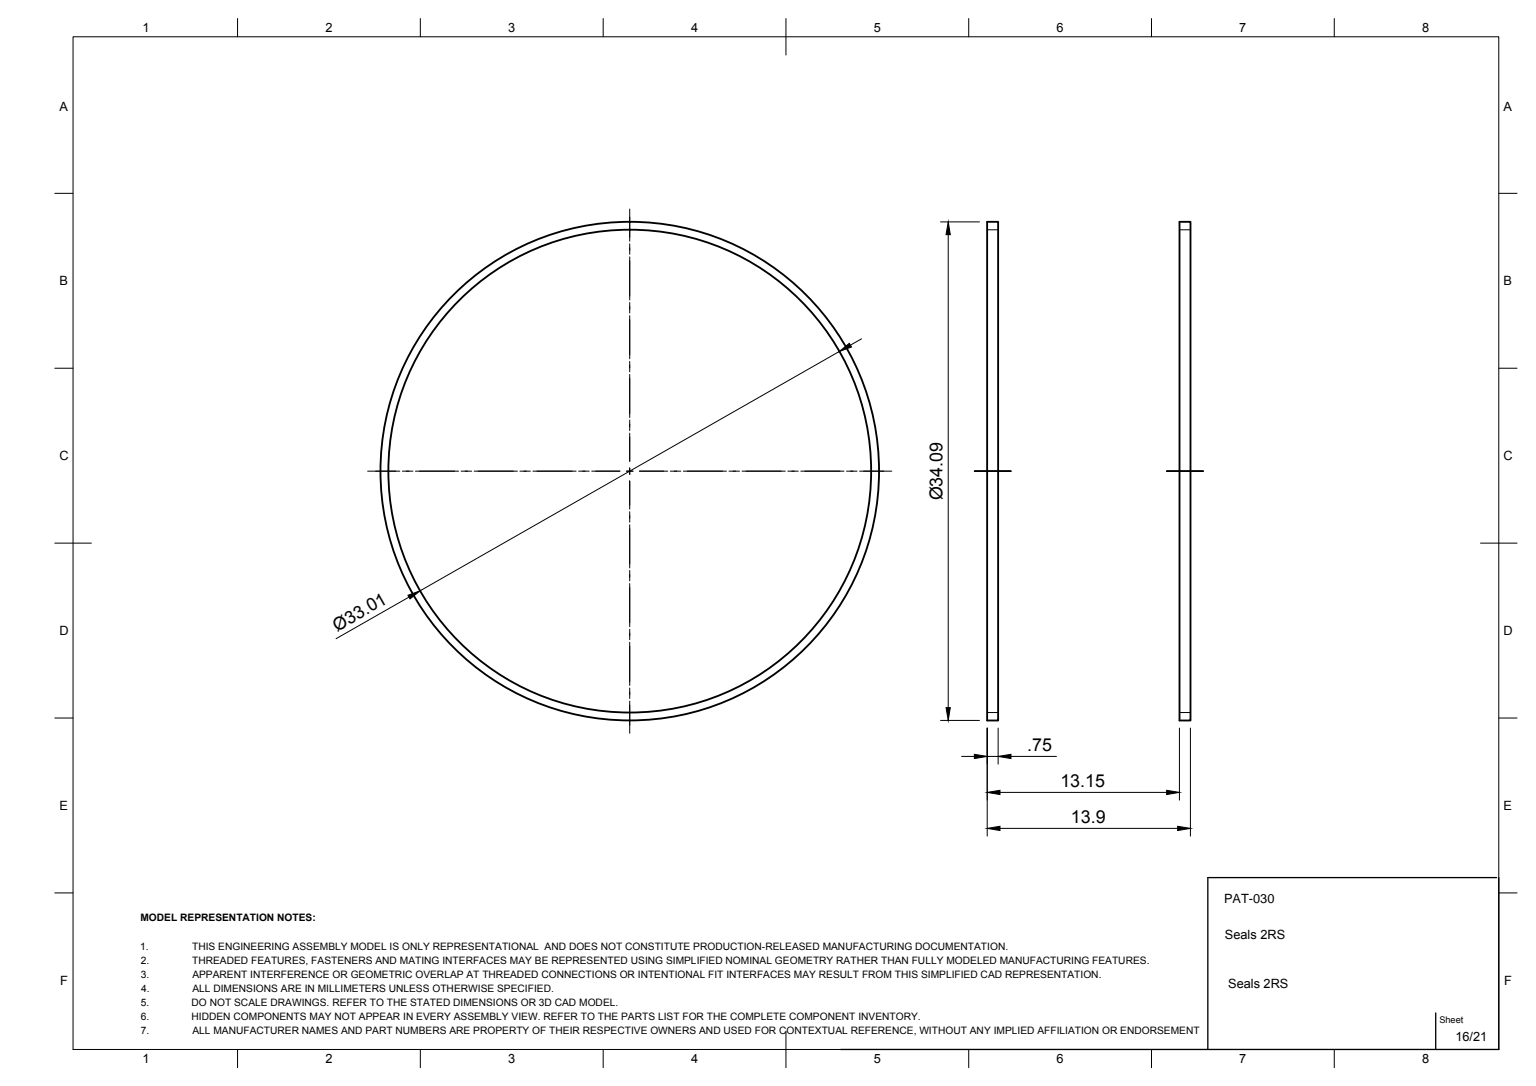
ISO-10303-21;
HEADER;
/* Generated by software containing ST-Developer
 * from STEP Tools, Inc. (www.steptools.com) 
 */

FILE_DESCRIPTION(
/* description */ ('Double-bearing flanged cartridge'),
/* implementation_level */ '2;1');

FILE_NAME(
/* name */ 'Seals 2RS.step',
/* time_stamp */ '2026-10-28T03:26:40-07:00',
/* author */ (''),
/* organization */ (''),
/* preprocessor_version */ 'ST-DEVELOPER v20.2',
/* originating_system */ 'Autodesk Translation Framework v15.17.0.0',
/* authorisation */ '');

FILE_SCHEMA (('AUTOMOTIVE_DESIGN { 1 0 10303 214 3 1 1 }'));
ENDSEC;

DATA;
#10=MECHANICAL_DESIGN_GEOMETRIC_PRESENTATION_REPRESENTATION('',(#202,#203),#5535);
#167=SHAPE_REPRESENTATION_RELATIONSHIP('SRR','None',#5609,#181);
#181=ADVANCED_BREP_SHAPE_REPRESENTATION('',(#224,#225),#5525);
#202=STYLED_ITEM('',(#5764),#224);
#203=STYLED_ITEM('',(#5764),#225);
#224=MANIFOLD_SOLID_BREP('Body1',#2336);
#225=MANIFOLD_SOLID_BREP('Body2',#2337);
#258=FACE_BOUND('',#607,.T.);
#259=FACE_BOUND('',#610,.T.);
#260=FACE_BOUND('',#613,.T.);
#261=FACE_BOUND('',#616,.T.);
#325=PLANE('',#2678);
#326=PLANE('',#2683);
#327=PLANE('',#2686);
#328=PLANE('',#2691);
#432=FACE_OUTER_BOUND('',#606,.T.);
#433=FACE_OUTER_BOUND('',#608,.T.);
#434=FACE_OUTER_BOUND('',#609,.T.);
#435=FACE_OUTER_BOUND('',#611,.T.);
#436=FACE_OUTER_BOUND('',#612,.T.);
#437=FACE_OUTER_BOUND('',#614,.T.);
#438=FACE_OUTER_BOUND('',#615,.T.);
#439=FACE_OUTER_BOUND('',#617,.T.);
#606=EDGE_LOOP('',(#1834));
#607=EDGE_LOOP('',(#1835));
#608=EDGE_LOOP('',(#1836,#1837,#1838,#1839));
#609=EDGE_LOOP('',(#1840));
#610=EDGE_LOOP('',(#1841));
#611=EDGE_LOOP('',(#1842,#1843,#1844,#1845));
#612=EDGE_LOOP('',(#1846));
#613=EDGE_LOOP('',(#1847));
#614=EDGE_LOOP('',(#1848,#1849,#1850,#1851));
#615=EDGE_LOOP('',(#1852));
#616=EDGE_LOOP('',(#1853));
#617=EDGE_LOOP('',(#1854,#1855,#1856,#1857));
#754=LINE('',#4355,#840);
#755=LINE('',#4360,#841);
#756=LINE('',#4369,#842);
#757=LINE('',#4374,#843);
#840=VECTOR('',#3257,1.70469);
#841=VECTOR('',#3264,1.65031);
#842=VECTOR('',#3275,1.70469);
#843=VECTOR('',#3282,1.65031);
#994=CIRCLE('',#2679,1.70469);
#995=CIRCLE('',#2680,1.65031);
#996=CIRCLE('',#2682,1.70469);
#997=CIRCLE('',#2684,1.65031);
#998=CIRCLE('',#2687,1.70469);
#999=CIRCLE('',#2688,1.65031);
#1000=CIRCLE('',#2690,1.70469);
#1001=CIRCLE('',#2692,1.65031);
#1176=VERTEX_POINT('',#4348);
#1177=VERTEX_POINT('',#4350);
#1178=VERTEX_POINT('',#4353);
#1179=VERTEX_POINT('',#4357);
#1180=VERTEX_POINT('',#4362);
#1181=VERTEX_POINT('',#4364);
#1182=VERTEX_POINT('',#4367);
#1183=VERTEX_POINT('',#4371);
#1410=EDGE_CURVE('',#1176,#1176,#994,.T.);
#1411=EDGE_CURVE('',#1177,#1177,#995,.T.);
#1412=EDGE_CURVE('',#1178,#1178,#996,.T.);
#1413=EDGE_CURVE('',#1178,#1176,#754,.T.);
#1414=EDGE_CURVE('',#1179,#1179,#997,.T.);
#1415=EDGE_CURVE('',#1179,#1177,#755,.T.);
#1416=EDGE_CURVE('',#1180,#1180,#998,.T.);
#1417=EDGE_CURVE('',#1181,#1181,#999,.T.);
#1418=EDGE_CURVE('',#1182,#1182,#1000,.T.);
#1419=EDGE_CURVE('',#1182,#1180,#756,.T.);
#1420=EDGE_CURVE('',#1183,#1183,#1001,.T.);
#1421=EDGE_CURVE('',#1183,#1181,#757,.T.);
#1834=ORIENTED_EDGE('',*,*,#1410,.F.);
#1835=ORIENTED_EDGE('',*,*,#1411,.T.);
#1836=ORIENTED_EDGE('',*,*,#1412,.F.);
#1837=ORIENTED_EDGE('',*,*,#1413,.T.);
#1838=ORIENTED_EDGE('',*,*,#1410,.T.);
#1839=ORIENTED_EDGE('',*,*,#1413,.F.);
#1840=ORIENTED_EDGE('',*,*,#1412,.T.);
#1841=ORIENTED_EDGE('',*,*,#1414,.F.);
#1842=ORIENTED_EDGE('',*,*,#1414,.T.);
#1843=ORIENTED_EDGE('',*,*,#1415,.T.);
#1844=ORIENTED_EDGE('',*,*,#1411,.F.);
#1845=ORIENTED_EDGE('',*,*,#1415,.F.);
#1846=ORIENTED_EDGE('',*,*,#1416,.F.);
#1847=ORIENTED_EDGE('',*,*,#1417,.T.);
#1848=ORIENTED_EDGE('',*,*,#1418,.F.);
#1849=ORIENTED_EDGE('',*,*,#1419,.T.);
#1850=ORIENTED_EDGE('',*,*,#1416,.T.);
#1851=ORIENTED_EDGE('',*,*,#1419,.F.);
#1852=ORIENTED_EDGE('',*,*,#1418,.T.);
#1853=ORIENTED_EDGE('',*,*,#1420,.F.);
#1854=ORIENTED_EDGE('',*,*,#1420,.T.);
#1855=ORIENTED_EDGE('',*,*,#1421,.T.);
#1856=ORIENTED_EDGE('',*,*,#1417,.F.);
#1857=ORIENTED_EDGE('',*,*,#1421,.F.);
#2138=CYLINDRICAL_SURFACE('',#2681,1.70469);
#2139=CYLINDRICAL_SURFACE('',#2685,1.65031);
#2140=CYLINDRICAL_SURFACE('',#2689,1.70469);
#2141=CYLINDRICAL_SURFACE('',#2693,1.65031);
#2246=ADVANCED_FACE('',(#432,#258),#325,.T.);
#2247=ADVANCED_FACE('',(#433),#2138,.T.);
#2248=ADVANCED_FACE('',(#434,#259),#326,.T.);
#2249=ADVANCED_FACE('',(#435),#2139,.F.);
#2250=ADVANCED_FACE('',(#436,#260),#327,.T.);
#2251=ADVANCED_FACE('',(#437),#2140,.T.);
#2252=ADVANCED_FACE('',(#438,#261),#328,.T.);
#2253=ADVANCED_FACE('',(#439),#2141,.F.);
#2336=CLOSED_SHELL('',(#2246,#2247,#2248,#2249));
#2337=CLOSED_SHELL('',(#2250,#2251,#2252,#2253));
#2677=AXIS2_PLACEMENT_3D('',#4346,#3245,#3246);
#2678=AXIS2_PLACEMENT_3D('',#4347,#3247,#3248);
#2679=AXIS2_PLACEMENT_3D('',#4349,#3249,#3250);
#2680=AXIS2_PLACEMENT_3D('',#4351,#3251,#3252);
#2681=AXIS2_PLACEMENT_3D('',#4352,#3253,#3254);
#2682=AXIS2_PLACEMENT_3D('',#4354,#3255,#3256);
#2683=AXIS2_PLACEMENT_3D('',#4356,#3258,#3259);
#2684=AXIS2_PLACEMENT_3D('',#4358,#3260,#3261);
#2685=AXIS2_PLACEMENT_3D('',#4359,#3262,#3263);
#2686=AXIS2_PLACEMENT_3D('',#4361,#3265,#3266);
#2687=AXIS2_PLACEMENT_3D('',#4363,#3267,#3268);
#2688=AXIS2_PLACEMENT_3D('',#4365,#3269,#3270);
#2689=AXIS2_PLACEMENT_3D('',#4366,#3271,#3272);
#2690=AXIS2_PLACEMENT_3D('',#4368,#3273,#3274);
#2691=AXIS2_PLACEMENT_3D('',#4370,#3276,#3277);
#2692=AXIS2_PLACEMENT_3D('',#4372,#3278,#3279);
#2693=AXIS2_PLACEMENT_3D('',#4373,#3280,#3281);
#3245=DIRECTION('axis',(0.,0.,1.));
#3246=DIRECTION('refdir',(1.,0.,0.));
#3247=DIRECTION('center_axis',(0.,1.,0.));
#3248=DIRECTION('ref_axis',(0.,0.,1.));
#3249=DIRECTION('center_axis',(0.,-1.,0.));
#3250=DIRECTION('ref_axis',(1.,0.,0.));
#3251=DIRECTION('center_axis',(0.,-1.,0.));
#3252=DIRECTION('ref_axis',(1.,0.,0.));
#3253=DIRECTION('center_axis',(0.,-1.,0.));
#3254=DIRECTION('ref_axis',(1.,0.,0.));
#3255=DIRECTION('center_axis',(0.,-1.,0.));
#3256=DIRECTION('ref_axis',(1.,0.,0.));
#3257=DIRECTION('',(0.,1.,0.));
#3258=DIRECTION('center_axis',(0.,-1.,0.));
#3259=DIRECTION('ref_axis',(0.,0.,-1.));
#3260=DIRECTION('center_axis',(0.,-1.,0.));
#3261=DIRECTION('ref_axis',(1.,0.,0.));
#3262=DIRECTION('center_axis',(0.,-1.,0.));
#3263=DIRECTION('ref_axis',(1.,0.,0.));
#3264=DIRECTION('',(0.,1.,0.));
#3265=DIRECTION('center_axis',(0.,1.,0.));
#3266=DIRECTION('ref_axis',(0.,0.,1.));
#3267=DIRECTION('center_axis',(0.,-1.,0.));
#3268=DIRECTION('ref_axis',(1.,0.,0.));
#3269=DIRECTION('center_axis',(0.,-1.,0.));
#3270=DIRECTION('ref_axis',(1.,0.,0.));
#3271=DIRECTION('center_axis',(0.,-1.,0.));
#3272=DIRECTION('ref_axis',(1.,0.,0.));
#3273=DIRECTION('center_axis',(0.,-1.,0.));
#3274=DIRECTION('ref_axis',(1.,0.,0.));
#3275=DIRECTION('',(0.,1.,0.));
#3276=DIRECTION('center_axis',(0.,-1.,0.));
#3277=DIRECTION('ref_axis',(0.,0.,-1.));
#3278=DIRECTION('center_axis',(0.,-1.,0.));
#3279=DIRECTION('ref_axis',(1.,0.,0.));
#3280=DIRECTION('center_axis',(0.,-1.,0.));
#3281=DIRECTION('ref_axis',(1.,0.,0.));
#3282=DIRECTION('',(0.,1.,0.));
#4346=CARTESIAN_POINT('',(0.,0.,0.));
#4347=CARTESIAN_POINT('Origin',(1.70469,0.695,0.));
#4348=CARTESIAN_POINT('',(-1.70469,0.695,-2.0876431520385E-16));
#4349=CARTESIAN_POINT('Origin',(0.,0.695,0.));
#4350=CARTESIAN_POINT('',(-1.65031,0.695,-2.02104685910087E-16));
#4351=CARTESIAN_POINT('Origin',(0.,0.695,0.));
#4352=CARTESIAN_POINT('Origin',(0.,0.6575,0.));
#4353=CARTESIAN_POINT('',(-1.70469,0.62,-2.0876431520385E-16));
#4354=CARTESIAN_POINT('Origin',(0.,0.62,0.));
#4355=CARTESIAN_POINT('',(-1.70469,0.6575,-2.0876431520385E-16));
#4356=CARTESIAN_POINT('Origin',(1.65031,0.62,0.));
#4357=CARTESIAN_POINT('',(-1.65031,0.62,-2.02104685910087E-16));
#4358=CARTESIAN_POINT('Origin',(0.,0.62,0.));
#4359=CARTESIAN_POINT('Origin',(0.,0.6575,0.));
#4360=CARTESIAN_POINT('',(-1.65031,0.6575,-2.02104685910087E-16));
#4361=CARTESIAN_POINT('Origin',(1.70469,-0.62,0.));
#4362=CARTESIAN_POINT('',(-1.70469,-0.62,-2.0876431520385E-16));
#4363=CARTESIAN_POINT('Origin',(0.,-0.62,0.));
#4364=CARTESIAN_POINT('',(-1.65031,-0.62,-2.02104685910087E-16));
#4365=CARTESIAN_POINT('Origin',(0.,-0.62,0.));
#4366=CARTESIAN_POINT('Origin',(0.,-0.6575,0.));
#4367=CARTESIAN_POINT('',(-1.70469,-0.695,-2.0876431520385E-16));
#4368=CARTESIAN_POINT('Origin',(0.,-0.695,0.));
#4369=CARTESIAN_POINT('',(-1.70469,-0.6575,-2.0876431520385E-16));
#4370=CARTESIAN_POINT('Origin',(1.65031,-0.695,0.));
#4371=CARTESIAN_POINT('',(-1.65031,-0.695,-2.02104685910087E-16));
#4372=CARTESIAN_POINT('Origin',(0.,-0.695,0.));
#4373=CARTESIAN_POINT('Origin',(0.,-0.6575,0.));
#4374=CARTESIAN_POINT('',(-1.65031,-0.6575,-2.02104685910087E-16));
#5506=UNCERTAINTY_MEASURE_WITH_UNIT(LENGTH_MEASURE(0.001),#5536,
'DISTANCE_ACCURACY_VALUE',
'Maximum model space distance between geometric entities at asserted c
onnectivities');
#5516=UNCERTAINTY_MEASURE_WITH_UNIT(LENGTH_MEASURE(0.001),#5536,
'DISTANCE_ACCURACY_VALUE',
'Maximum model space distance between geometric entities at asserted c
onnectivities');
#5525=(
GEOMETRIC_REPRESENTATION_CONTEXT(3)
GLOBAL_UNCERTAINTY_ASSIGNED_CONTEXT((#5506))
GLOBAL_UNIT_ASSIGNED_CONTEXT((#5536,#5538,#5539))
REPRESENTATION_CONTEXT('','3D')
);
#5535=(
GEOMETRIC_REPRESENTATION_CONTEXT(3)
GLOBAL_UNCERTAINTY_ASSIGNED_CONTEXT((#5516))
GLOBAL_UNIT_ASSIGNED_CONTEXT((#5536,#5538,#5539))
REPRESENTATION_CONTEXT('','3D')
);
#5536=(
LENGTH_UNIT()
NAMED_UNIT(*)
SI_UNIT(.CENTI.,.METRE.)
);
#5538=(
NAMED_UNIT(*)
PLANE_ANGLE_UNIT()
SI_UNIT($,.RADIAN.)
);
#5539=(
NAMED_UNIT(*)
SI_UNIT($,.STERADIAN.)
SOLID_ANGLE_UNIT()
);
#5548=SHAPE_DEFINITION_REPRESENTATION(#5566,#5609);
#5566=PRODUCT_DEFINITION_SHAPE('',$,#5628);
#5609=SHAPE_REPRESENTATION('',(#2677),#5525);
#5619=PRODUCT_DEFINITION_CONTEXT('part definition',#5675,'design');
#5628=PRODUCT_DEFINITION('Seals 2RS','Seals 2RS',#5646,#5619);
#5646=PRODUCT_DEFINITION_FORMATION('',$,#5685);
#5675=APPLICATION_CONTEXT(
'Core Data for Automotive Mechanical Design Process');
#5676=PRODUCT_CONTEXT('part definition',#5675,'mechanical');
#5685=PRODUCT('Seals 2RS','Seals 2RS','Seals 2RS',(#5676));
#5758=COLOUR_RGB('Grey',0.48,0.52,0.57);
#5759=FILL_AREA_STYLE_COLOUR('',#5758);
#5760=FILL_AREA_STYLE('',(#5759));
#5761=SURFACE_STYLE_FILL_AREA(#5760);
#5762=SURFACE_SIDE_STYLE('',(#5761));
#5763=SURFACE_STYLE_USAGE(.BOTH.,#5762);
#5764=PRESENTATION_STYLE_ASSIGNMENT((#5763));
ENDSEC;
END-ISO-10303-21;
